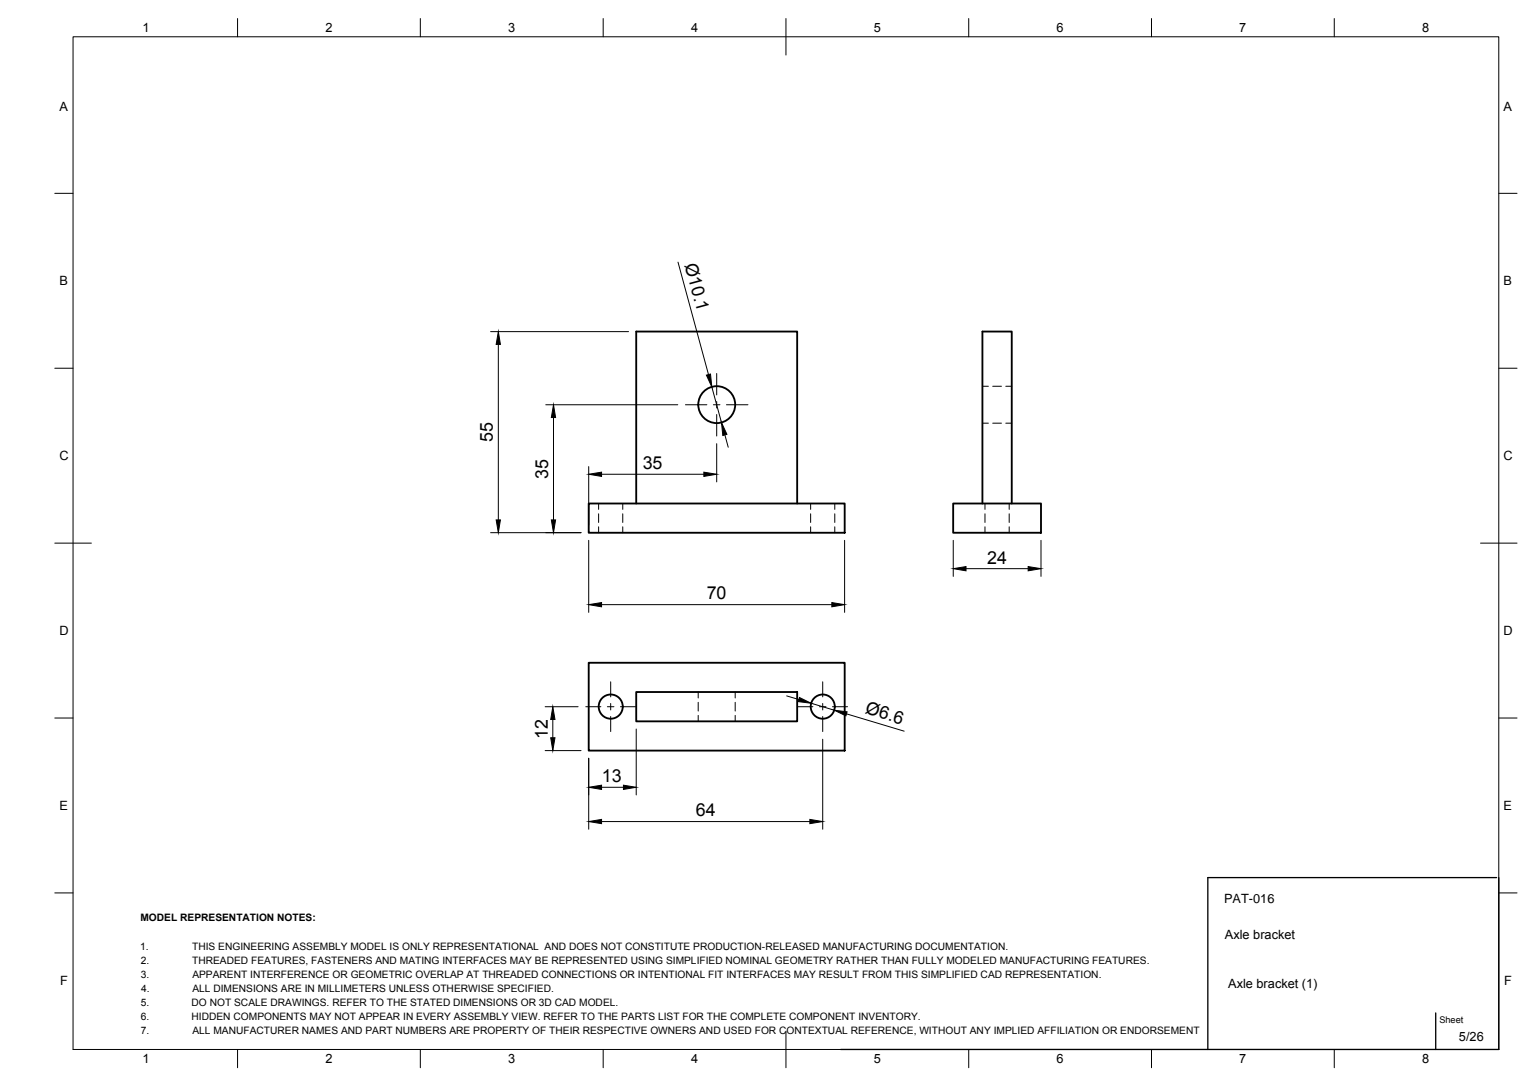
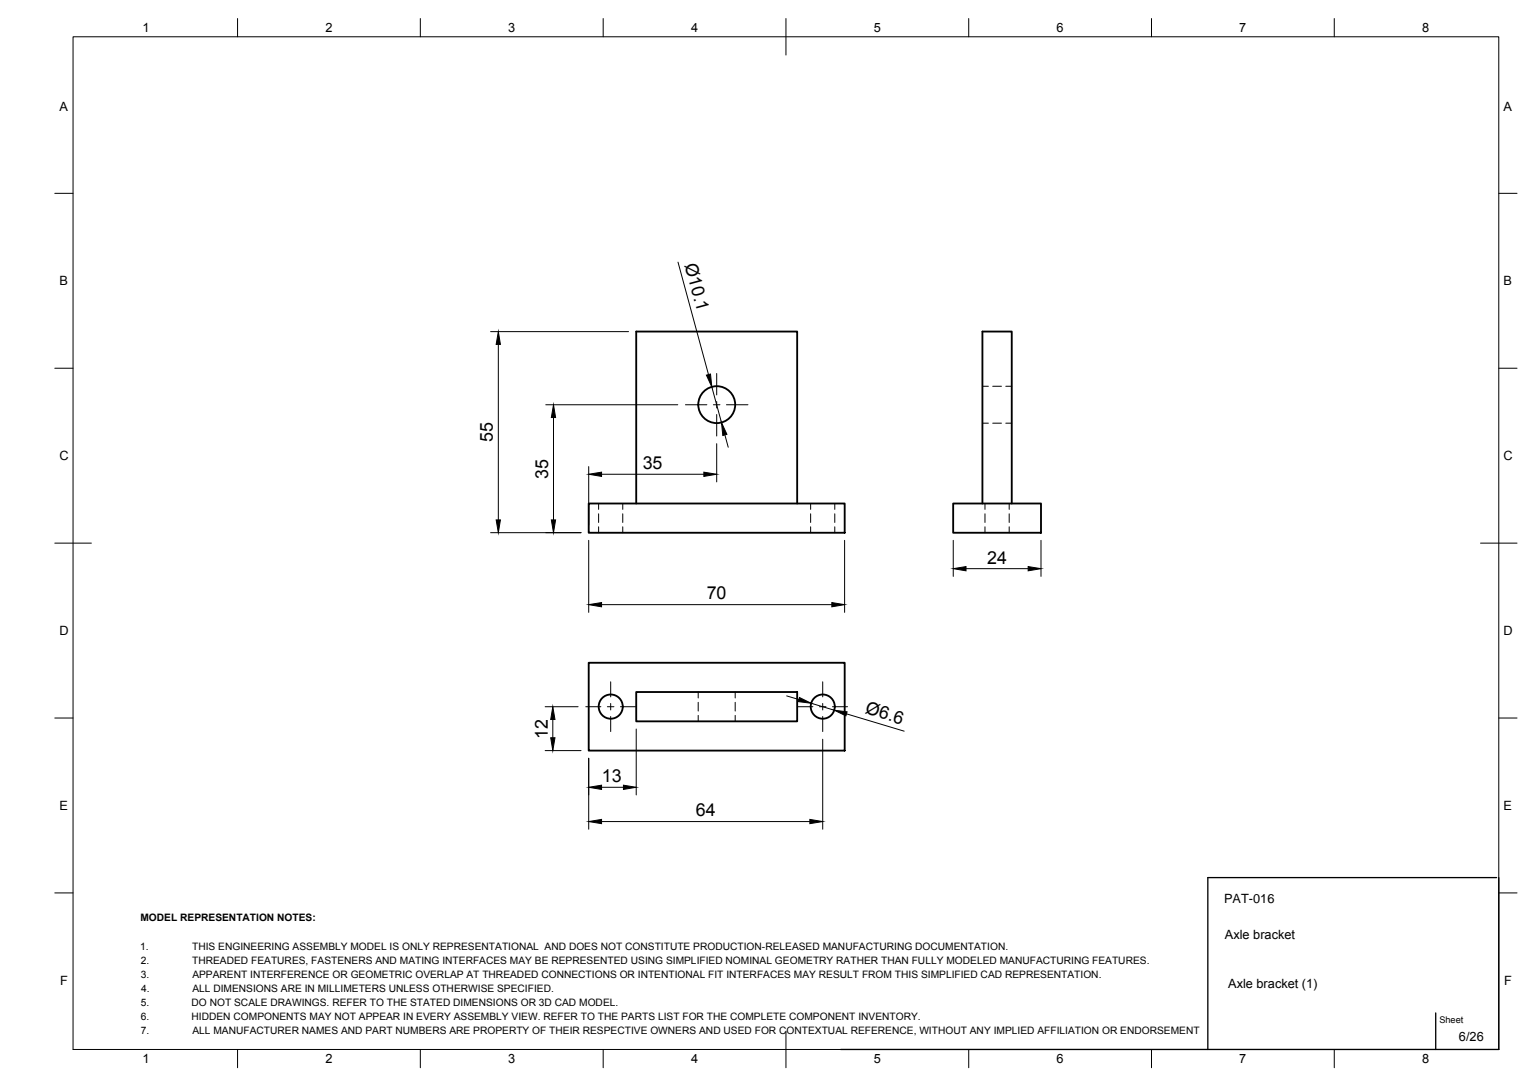
ISO-10303-21;
HEADER;
/* Generated by software containing ST-Developer
 * from STEP Tools, Inc. (www.steptools.com) 
 */

FILE_DESCRIPTION(
/* description */ ('Bracket-mounted idler roller'),
/* implementation_level */ '2;1');

FILE_NAME(
/* name */ 'Axle bracket (1).step',
/* time_stamp */ '2026-10-28T03:26:42-07:00',
/* author */ (''),
/* organization */ (''),
/* preprocessor_version */ 'ST-DEVELOPER v20.2',
/* originating_system */ 'Autodesk Translation Framework v15.17.0.0',
/* authorisation */ '');

FILE_SCHEMA (('AUTOMOTIVE_DESIGN { 1 0 10303 214 3 1 1 }'));
ENDSEC;

DATA;
#10=MECHANICAL_DESIGN_GEOMETRIC_PRESENTATION_REPRESENTATION('',(#281),#6241);
#239=SHAPE_REPRESENTATION_RELATIONSHIP('SRR','None',#6343,#260);
#260=ADVANCED_BREP_SHAPE_REPRESENTATION('',(#310),#6219);
#281=STYLED_ITEM('',(#6538),#310);
#310=MANIFOLD_SOLID_BREP('Body1',#3183);
#343=FACE_BOUND('',#732,.T.);
#344=FACE_BOUND('',#733,.T.);
#345=FACE_BOUND('',#734,.T.);
#346=FACE_BOUND('',#740,.T.);
#347=FACE_BOUND('',#743,.T.);
#348=FACE_BOUND('',#747,.T.);
#349=FACE_BOUND('',#748,.T.);
#428=PLANE('',#3478);
#429=PLANE('',#3479);
#430=PLANE('',#3480);
#431=PLANE('',#3481);
#432=PLANE('',#3482);
#433=PLANE('',#3483);
#434=PLANE('',#3484);
#435=PLANE('',#3485);
#436=PLANE('',#3486);
#437=PLANE('',#3487);
#438=PLANE('',#3488);
#530=FACE_OUTER_BOUND('',#728,.T.);
#531=FACE_OUTER_BOUND('',#729,.T.);
#532=FACE_OUTER_BOUND('',#730,.T.);
#533=FACE_OUTER_BOUND('',#731,.T.);
#534=FACE_OUTER_BOUND('',#735,.T.);
#535=FACE_OUTER_BOUND('',#736,.T.);
#536=FACE_OUTER_BOUND('',#737,.T.);
#537=FACE_OUTER_BOUND('',#738,.T.);
#538=FACE_OUTER_BOUND('',#739,.T.);
#539=FACE_OUTER_BOUND('',#741,.T.);
#540=FACE_OUTER_BOUND('',#742,.T.);
#541=FACE_OUTER_BOUND('',#744,.T.);
#542=FACE_OUTER_BOUND('',#745,.T.);
#543=FACE_OUTER_BOUND('',#746,.T.);
#728=EDGE_LOOP('',(#2232,#2233,#2234,#2235));
#729=EDGE_LOOP('',(#2236,#2237,#2238,#2239));
#730=EDGE_LOOP('',(#2240,#2241,#2242,#2243));
#731=EDGE_LOOP('',(#2244,#2245,#2246,#2247));
#732=EDGE_LOOP('',(#2248));
#733=EDGE_LOOP('',(#2249));
#734=EDGE_LOOP('',(#2250,#2251,#2252,#2253));
#735=EDGE_LOOP('',(#2254,#2255,#2256,#2257));
#736=EDGE_LOOP('',(#2258,#2259,#2260,#2261));
#737=EDGE_LOOP('',(#2262,#2263,#2264,#2265));
#738=EDGE_LOOP('',(#2266,#2267,#2268,#2269));
#739=EDGE_LOOP('',(#2270,#2271,#2272,#2273));
#740=EDGE_LOOP('',(#2274));
#741=EDGE_LOOP('',(#2275,#2276,#2277,#2278));
#742=EDGE_LOOP('',(#2279,#2280,#2281,#2282));
#743=EDGE_LOOP('',(#2283));
#744=EDGE_LOOP('',(#2284,#2285,#2286,#2287));
#745=EDGE_LOOP('',(#2288,#2289,#2290,#2291));
#746=EDGE_LOOP('',(#2292,#2293,#2294,#2295));
#747=EDGE_LOOP('',(#2296));
#748=EDGE_LOOP('',(#2297));
#1006=LINE('',#5027,#1188);
#1007=LINE('',#5033,#1189);
#1008=LINE('',#5039,#1190);
#1009=LINE('',#5044,#1191);
#1010=LINE('',#5046,#1192);
#1011=LINE('',#5048,#1193);
#1012=LINE('',#5049,#1194);
#1013=LINE('',#5052,#1195);
#1014=LINE('',#5054,#1196);
#1015=LINE('',#5056,#1197);
#1016=LINE('',#5057,#1198);
#1017=LINE('',#5060,#1199);
#1018=LINE('',#5062,#1200);
#1019=LINE('',#5063,#1201);
#1020=LINE('',#5066,#1202);
#1021=LINE('',#5068,#1203);
#1022=LINE('',#5069,#1204);
#1023=LINE('',#5071,#1205);
#1024=LINE('',#5073,#1206);
#1025=LINE('',#5076,#1207);
#1026=LINE('',#5078,#1208);
#1027=LINE('',#5079,#1209);
#1028=LINE('',#5082,#1210);
#1029=LINE('',#5083,#1211);
#1030=LINE('',#5086,#1212);
#1031=LINE('',#5087,#1213);
#1032=LINE('',#5089,#1214);
#1188=VECTOR('',#3965,0.33);
#1189=VECTOR('',#3972,0.33);
#1190=VECTOR('',#3979,0.505);
#1191=VECTOR('',#3984,1.);
#1192=VECTOR('',#3985,1.);
#1193=VECTOR('',#3986,1.);
#1194=VECTOR('',#3987,1.);
#1195=VECTOR('',#3988,1.);
#1196=VECTOR('',#3989,1.);
#1197=VECTOR('',#3990,1.);
#1198=VECTOR('',#3991,1.);
#1199=VECTOR('',#3994,1.);
#1200=VECTOR('',#3995,1.);
#1201=VECTOR('',#3996,1.);
#1202=VECTOR('',#3999,1.);
#1203=VECTOR('',#4000,1.);
#1204=VECTOR('',#4001,1.);
#1205=VECTOR('',#4004,1.);
#1206=VECTOR('',#4007,1.);
#1207=VECTOR('',#4010,1.);
#1208=VECTOR('',#4011,1.);
#1209=VECTOR('',#4012,1.);
#1210=VECTOR('',#4015,1.);
#1211=VECTOR('',#4016,1.);
#1212=VECTOR('',#4019,1.);
#1213=VECTOR('',#4020,1.);
#1214=VECTOR('',#4023,1.);
#1349=CIRCLE('',#3470,0.33);
#1350=CIRCLE('',#3471,0.33);
#1351=CIRCLE('',#3473,0.33);
#1352=CIRCLE('',#3474,0.33);
#1353=CIRCLE('',#3476,0.505);
#1354=CIRCLE('',#3477,0.505);
#1546=VERTEX_POINT('',#5024);
#1547=VERTEX_POINT('',#5026);
#1548=VERTEX_POINT('',#5030);
#1549=VERTEX_POINT('',#5032);
#1550=VERTEX_POINT('',#5036);
#1551=VERTEX_POINT('',#5038);
#1552=VERTEX_POINT('',#5042);
#1553=VERTEX_POINT('',#5043);
#1554=VERTEX_POINT('',#5045);
#1555=VERTEX_POINT('',#5047);
#1556=VERTEX_POINT('',#5050);
#1557=VERTEX_POINT('',#5051);
#1558=VERTEX_POINT('',#5053);
#1559=VERTEX_POINT('',#5055);
#1560=VERTEX_POINT('',#5059);
#1561=VERTEX_POINT('',#5061);
#1562=VERTEX_POINT('',#5065);
#1563=VERTEX_POINT('',#5067);
#1564=VERTEX_POINT('',#5075);
#1565=VERTEX_POINT('',#5077);
#1566=VERTEX_POINT('',#5081);
#1567=VERTEX_POINT('',#5085);
#1818=EDGE_CURVE('',#1546,#1546,#1349,.T.);
#1819=EDGE_CURVE('',#1546,#1547,#1006,.T.);
#1820=EDGE_CURVE('',#1547,#1547,#1350,.T.);
#1821=EDGE_CURVE('',#1548,#1548,#1351,.T.);
#1822=EDGE_CURVE('',#1548,#1549,#1007,.T.);
#1823=EDGE_CURVE('',#1549,#1549,#1352,.T.);
#1824=EDGE_CURVE('',#1550,#1550,#1353,.T.);
#1825=EDGE_CURVE('',#1550,#1551,#1008,.T.);
#1826=EDGE_CURVE('',#1551,#1551,#1354,.T.);
#1827=EDGE_CURVE('',#1552,#1553,#1009,.T.);
#1828=EDGE_CURVE('',#1552,#1554,#1010,.T.);
#1829=EDGE_CURVE('',#1555,#1554,#1011,.T.);
#1830=EDGE_CURVE('',#1553,#1555,#1012,.T.);
#1831=EDGE_CURVE('',#1556,#1557,#1013,.T.);
#1832=EDGE_CURVE('',#1558,#1556,#1014,.T.);
#1833=EDGE_CURVE('',#1559,#1558,#1015,.T.);
#1834=EDGE_CURVE('',#1557,#1559,#1016,.T.);
#1835=EDGE_CURVE('',#1553,#1560,#1017,.T.);
#1836=EDGE_CURVE('',#1561,#1555,#1018,.T.);
#1837=EDGE_CURVE('',#1560,#1561,#1019,.T.);
#1838=EDGE_CURVE('',#1562,#1552,#1020,.T.);
#1839=EDGE_CURVE('',#1562,#1563,#1021,.T.);
#1840=EDGE_CURVE('',#1554,#1563,#1022,.T.);
#1841=EDGE_CURVE('',#1563,#1561,#1023,.T.);
#1842=EDGE_CURVE('',#1560,#1562,#1024,.T.);
#1843=EDGE_CURVE('',#1558,#1564,#1025,.T.);
#1844=EDGE_CURVE('',#1565,#1564,#1026,.T.);
#1845=EDGE_CURVE('',#1559,#1565,#1027,.T.);
#1846=EDGE_CURVE('',#1556,#1566,#1028,.T.);
#1847=EDGE_CURVE('',#1564,#1566,#1029,.T.);
#1848=EDGE_CURVE('',#1557,#1567,#1030,.T.);
#1849=EDGE_CURVE('',#1566,#1567,#1031,.T.);
#1850=EDGE_CURVE('',#1567,#1565,#1032,.T.);
#2232=ORIENTED_EDGE('',*,*,#1818,.F.);
#2233=ORIENTED_EDGE('',*,*,#1819,.T.);
#2234=ORIENTED_EDGE('',*,*,#1820,.F.);
#2235=ORIENTED_EDGE('',*,*,#1819,.F.);
#2236=ORIENTED_EDGE('',*,*,#1821,.F.);
#2237=ORIENTED_EDGE('',*,*,#1822,.T.);
#2238=ORIENTED_EDGE('',*,*,#1823,.F.);
#2239=ORIENTED_EDGE('',*,*,#1822,.F.);
#2240=ORIENTED_EDGE('',*,*,#1824,.F.);
#2241=ORIENTED_EDGE('',*,*,#1825,.T.);
#2242=ORIENTED_EDGE('',*,*,#1826,.F.);
#2243=ORIENTED_EDGE('',*,*,#1825,.F.);
#2244=ORIENTED_EDGE('',*,*,#1827,.F.);
#2245=ORIENTED_EDGE('',*,*,#1828,.T.);
#2246=ORIENTED_EDGE('',*,*,#1829,.F.);
#2247=ORIENTED_EDGE('',*,*,#1830,.F.);
#2248=ORIENTED_EDGE('',*,*,#1820,.T.);
#2249=ORIENTED_EDGE('',*,*,#1823,.T.);
#2250=ORIENTED_EDGE('',*,*,#1831,.F.);
#2251=ORIENTED_EDGE('',*,*,#1832,.F.);
#2252=ORIENTED_EDGE('',*,*,#1833,.F.);
#2253=ORIENTED_EDGE('',*,*,#1834,.F.);
#2254=ORIENTED_EDGE('',*,*,#1835,.F.);
#2255=ORIENTED_EDGE('',*,*,#1830,.T.);
#2256=ORIENTED_EDGE('',*,*,#1836,.F.);
#2257=ORIENTED_EDGE('',*,*,#1837,.F.);
#2258=ORIENTED_EDGE('',*,*,#1838,.F.);
#2259=ORIENTED_EDGE('',*,*,#1839,.T.);
#2260=ORIENTED_EDGE('',*,*,#1840,.F.);
#2261=ORIENTED_EDGE('',*,*,#1828,.F.);
#2262=ORIENTED_EDGE('',*,*,#1829,.T.);
#2263=ORIENTED_EDGE('',*,*,#1840,.T.);
#2264=ORIENTED_EDGE('',*,*,#1841,.T.);
#2265=ORIENTED_EDGE('',*,*,#1836,.T.);
#2266=ORIENTED_EDGE('',*,*,#1827,.T.);
#2267=ORIENTED_EDGE('',*,*,#1835,.T.);
#2268=ORIENTED_EDGE('',*,*,#1842,.T.);
#2269=ORIENTED_EDGE('',*,*,#1838,.T.);
#2270=ORIENTED_EDGE('',*,*,#1833,.T.);
#2271=ORIENTED_EDGE('',*,*,#1843,.T.);
#2272=ORIENTED_EDGE('',*,*,#1844,.F.);
#2273=ORIENTED_EDGE('',*,*,#1845,.F.);
#2274=ORIENTED_EDGE('',*,*,#1824,.T.);
#2275=ORIENTED_EDGE('',*,*,#1832,.T.);
#2276=ORIENTED_EDGE('',*,*,#1846,.T.);
#2277=ORIENTED_EDGE('',*,*,#1847,.F.);
#2278=ORIENTED_EDGE('',*,*,#1843,.F.);
#2279=ORIENTED_EDGE('',*,*,#1831,.T.);
#2280=ORIENTED_EDGE('',*,*,#1848,.T.);
#2281=ORIENTED_EDGE('',*,*,#1849,.F.);
#2282=ORIENTED_EDGE('',*,*,#1846,.F.);
#2283=ORIENTED_EDGE('',*,*,#1826,.T.);
#2284=ORIENTED_EDGE('',*,*,#1834,.T.);
#2285=ORIENTED_EDGE('',*,*,#1845,.T.);
#2286=ORIENTED_EDGE('',*,*,#1850,.F.);
#2287=ORIENTED_EDGE('',*,*,#1848,.F.);
#2288=ORIENTED_EDGE('',*,*,#1850,.T.);
#2289=ORIENTED_EDGE('',*,*,#1844,.T.);
#2290=ORIENTED_EDGE('',*,*,#1847,.T.);
#2291=ORIENTED_EDGE('',*,*,#1849,.T.);
#2292=ORIENTED_EDGE('',*,*,#1842,.F.);
#2293=ORIENTED_EDGE('',*,*,#1837,.T.);
#2294=ORIENTED_EDGE('',*,*,#1841,.F.);
#2295=ORIENTED_EDGE('',*,*,#1839,.F.);
#2296=ORIENTED_EDGE('',*,*,#1818,.T.);
#2297=ORIENTED_EDGE('',*,*,#1821,.T.);
#2931=CYLINDRICAL_SURFACE('',#3469,0.33);
#2932=CYLINDRICAL_SURFACE('',#3472,0.33);
#2933=CYLINDRICAL_SURFACE('',#3475,0.505);
#3005=ADVANCED_FACE('',(#530),#2931,.F.);
#3006=ADVANCED_FACE('',(#531),#2932,.F.);
#3007=ADVANCED_FACE('',(#532),#2933,.F.);
#3008=ADVANCED_FACE('',(#533,#343,#344,#345),#428,.T.);
#3009=ADVANCED_FACE('',(#534),#429,.T.);
#3010=ADVANCED_FACE('',(#535),#430,.T.);
#3011=ADVANCED_FACE('',(#536),#431,.T.);
#3012=ADVANCED_FACE('',(#537),#432,.F.);
#3013=ADVANCED_FACE('',(#538,#346),#433,.T.);
#3014=ADVANCED_FACE('',(#539),#434,.T.);
#3015=ADVANCED_FACE('',(#540,#347),#435,.T.);
#3016=ADVANCED_FACE('',(#541),#436,.T.);
#3017=ADVANCED_FACE('',(#542),#437,.T.);
#3018=ADVANCED_FACE('',(#543,#348,#349),#438,.F.);
#3183=CLOSED_SHELL('',(#3005,#3006,#3007,#3008,#3009,#3010,#3011,#3012,
#3013,#3014,#3015,#3016,#3017,#3018));
#3468=AXIS2_PLACEMENT_3D('',#5022,#3959,#3960);
#3469=AXIS2_PLACEMENT_3D('',#5023,#3961,#3962);
#3470=AXIS2_PLACEMENT_3D('',#5025,#3963,#3964);
#3471=AXIS2_PLACEMENT_3D('',#5028,#3966,#3967);
#3472=AXIS2_PLACEMENT_3D('',#5029,#3968,#3969);
#3473=AXIS2_PLACEMENT_3D('',#5031,#3970,#3971);
#3474=AXIS2_PLACEMENT_3D('',#5034,#3973,#3974);
#3475=AXIS2_PLACEMENT_3D('',#5035,#3975,#3976);
#3476=AXIS2_PLACEMENT_3D('',#5037,#3977,#3978);
#3477=AXIS2_PLACEMENT_3D('',#5040,#3980,#3981);
#3478=AXIS2_PLACEMENT_3D('',#5041,#3982,#3983);
#3479=AXIS2_PLACEMENT_3D('',#5058,#3992,#3993);
#3480=AXIS2_PLACEMENT_3D('',#5064,#3997,#3998);
#3481=AXIS2_PLACEMENT_3D('',#5070,#4002,#4003);
#3482=AXIS2_PLACEMENT_3D('',#5072,#4005,#4006);
#3483=AXIS2_PLACEMENT_3D('',#5074,#4008,#4009);
#3484=AXIS2_PLACEMENT_3D('',#5080,#4013,#4014);
#3485=AXIS2_PLACEMENT_3D('',#5084,#4017,#4018);
#3486=AXIS2_PLACEMENT_3D('',#5088,#4021,#4022);
#3487=AXIS2_PLACEMENT_3D('',#5090,#4024,#4025);
#3488=AXIS2_PLACEMENT_3D('',#5091,#4026,#4027);
#3959=DIRECTION('axis',(0.,0.,1.));
#3960=DIRECTION('refdir',(1.,0.,0.));
#3961=DIRECTION('center_axis',(0.,0.,1.));
#3962=DIRECTION('ref_axis',(1.,0.,0.));
#3963=DIRECTION('center_axis',(0.,0.,1.));
#3964=DIRECTION('ref_axis',(1.,0.,0.));
#3965=DIRECTION('',(0.,0.,1.));
#3966=DIRECTION('center_axis',(0.,0.,-1.));
#3967=DIRECTION('ref_axis',(1.,0.,0.));
#3968=DIRECTION('center_axis',(0.,0.,1.));
#3969=DIRECTION('ref_axis',(1.,0.,0.));
#3970=DIRECTION('center_axis',(0.,0.,1.));
#3971=DIRECTION('ref_axis',(1.,0.,0.));
#3972=DIRECTION('',(0.,0.,1.));
#3973=DIRECTION('center_axis',(0.,0.,-1.));
#3974=DIRECTION('ref_axis',(1.,0.,0.));
#3975=DIRECTION('center_axis',(0.,1.,0.));
#3976=DIRECTION('ref_axis',(1.,0.,0.));
#3977=DIRECTION('center_axis',(0.,1.,0.));
#3978=DIRECTION('ref_axis',(1.,0.,0.));
#3979=DIRECTION('',(0.,1.,0.));
#3980=DIRECTION('center_axis',(0.,-1.,0.));
#3981=DIRECTION('ref_axis',(1.,0.,0.));
#3982=DIRECTION('center_axis',(0.,0.,1.));
#3983=DIRECTION('ref_axis',(1.,0.,0.));
#3984=DIRECTION('',(-1.,0.,0.));
#3985=DIRECTION('',(0.,1.,0.));
#3986=DIRECTION('',(1.,0.,0.));
#3987=DIRECTION('',(0.,1.,0.));
#3988=DIRECTION('',(-1.,0.,0.));
#3989=DIRECTION('',(0.,1.,0.));
#3990=DIRECTION('',(1.,0.,0.));
#3991=DIRECTION('',(0.,-1.,0.));
#3992=DIRECTION('center_axis',(-1.,0.,0.));
#3993=DIRECTION('ref_axis',(0.,0.,1.));
#3994=DIRECTION('',(0.,0.,-1.));
#3995=DIRECTION('',(0.,0.,1.));
#3996=DIRECTION('',(0.,1.,0.));
#3997=DIRECTION('center_axis',(1.,0.,0.));
#3998=DIRECTION('ref_axis',(0.,0.,-1.));
#3999=DIRECTION('',(0.,0.,1.));
#4000=DIRECTION('',(0.,1.,0.));
#4001=DIRECTION('',(0.,0.,-1.));
#4002=DIRECTION('center_axis',(0.,1.,0.));
#4003=DIRECTION('ref_axis',(0.,0.,1.));
#4004=DIRECTION('',(-1.,0.,0.));
#4005=DIRECTION('center_axis',(0.,1.,0.));
#4006=DIRECTION('ref_axis',(1.,0.,0.));
#4007=DIRECTION('',(1.,0.,0.));
#4008=DIRECTION('center_axis',(0.,-1.,0.));
#4009=DIRECTION('ref_axis',(1.,0.,0.));
#4010=DIRECTION('',(0.,0.,1.));
#4011=DIRECTION('',(1.,0.,0.));
#4012=DIRECTION('',(0.,0.,1.));
#4013=DIRECTION('center_axis',(1.,0.,0.));
#4014=DIRECTION('ref_axis',(0.,1.,0.));
#4015=DIRECTION('',(0.,0.,1.));
#4016=DIRECTION('',(0.,1.,0.));
#4017=DIRECTION('center_axis',(0.,1.,0.));
#4018=DIRECTION('ref_axis',(-1.,0.,0.));
#4019=DIRECTION('',(0.,0.,1.));
#4020=DIRECTION('',(-1.,0.,0.));
#4021=DIRECTION('center_axis',(-1.,0.,0.));
#4022=DIRECTION('ref_axis',(0.,-1.,0.));
#4023=DIRECTION('',(0.,-1.,0.));
#4024=DIRECTION('center_axis',(0.,0.,1.));
#4025=DIRECTION('ref_axis',(1.,0.,0.));
#4026=DIRECTION('center_axis',(0.,0.,1.));
#4027=DIRECTION('ref_axis',(1.,0.,0.));
#5022=CARTESIAN_POINT('',(0.,0.,0.));
#5023=CARTESIAN_POINT('Origin',(-2.9,32.,0.9));
#5024=CARTESIAN_POINT('',(-3.23,32.,1.));
#5025=CARTESIAN_POINT('Origin',(-2.9,32.,1.));
#5026=CARTESIAN_POINT('',(-3.23,32.,1.8));
#5027=CARTESIAN_POINT('',(-3.23,32.,0.9));
#5028=CARTESIAN_POINT('Origin',(-2.9,32.,1.8));
#5029=CARTESIAN_POINT('Origin',(2.9,32.,0.9));
#5030=CARTESIAN_POINT('',(2.57,32.,1.));
#5031=CARTESIAN_POINT('Origin',(2.9,32.,1.));
#5032=CARTESIAN_POINT('',(2.57,32.,1.8));
#5033=CARTESIAN_POINT('',(2.57,32.,0.9));
#5034=CARTESIAN_POINT('Origin',(2.9,32.,1.8));
#5035=CARTESIAN_POINT('Origin',(0.,31.5,4.5));
#5036=CARTESIAN_POINT('',(-0.505,31.6,4.5));
#5037=CARTESIAN_POINT('Origin',(0.,31.6,4.5));
#5038=CARTESIAN_POINT('',(-0.505,32.4,4.5));
#5039=CARTESIAN_POINT('',(-0.505,31.5,4.5));
#5040=CARTESIAN_POINT('Origin',(0.,32.4,4.5));
#5041=CARTESIAN_POINT('Origin',(-3.5,30.8,1.8));
#5042=CARTESIAN_POINT('',(3.5,30.8,1.8));
#5043=CARTESIAN_POINT('',(-3.5,30.8,1.8));
#5044=CARTESIAN_POINT('',(3.5,30.8,1.8));
#5045=CARTESIAN_POINT('',(3.5,33.2,1.8));
#5046=CARTESIAN_POINT('',(3.5,30.8,1.8));
#5047=CARTESIAN_POINT('',(-3.5,33.2,1.8));
#5048=CARTESIAN_POINT('',(3.5,33.2,1.8));
#5049=CARTESIAN_POINT('',(-3.5,30.8,1.8));
#5050=CARTESIAN_POINT('',(2.2,32.4,1.8));
#5051=CARTESIAN_POINT('',(-2.2,32.4,1.8));
#5052=CARTESIAN_POINT('',(-0.65,32.4,1.8));
#5053=CARTESIAN_POINT('',(2.2,31.6,1.8));
#5054=CARTESIAN_POINT('',(2.2,31.2,1.8));
#5055=CARTESIAN_POINT('',(-2.2,31.6,1.8));
#5056=CARTESIAN_POINT('',(-2.85,31.6,1.8));
#5057=CARTESIAN_POINT('',(-2.2,31.6,1.8));
#5058=CARTESIAN_POINT('Origin',(-3.5,30.8,1.));
#5059=CARTESIAN_POINT('',(-3.5,30.8,1.));
#5060=CARTESIAN_POINT('',(-3.5,30.8,1.8));
#5061=CARTESIAN_POINT('',(-3.5,33.2,1.));
#5062=CARTESIAN_POINT('',(-3.5,33.2,1.8));
#5063=CARTESIAN_POINT('',(-3.5,30.8,1.));
#5064=CARTESIAN_POINT('Origin',(3.5,30.8,1.8));
#5065=CARTESIAN_POINT('',(3.5,30.8,1.));
#5066=CARTESIAN_POINT('',(3.5,30.8,1.));
#5067=CARTESIAN_POINT('',(3.5,33.2,1.));
#5068=CARTESIAN_POINT('',(3.5,30.8,1.));
#5069=CARTESIAN_POINT('',(3.5,33.2,1.));
#5070=CARTESIAN_POINT('Origin',(0.,33.2,1.4));
#5071=CARTESIAN_POINT('',(-3.5,33.2,1.));
#5072=CARTESIAN_POINT('Origin',(0.,30.8,1.4));
#5073=CARTESIAN_POINT('',(-3.5,30.8,1.));
#5074=CARTESIAN_POINT('Origin',(-2.2,31.6,1.));
#5075=CARTESIAN_POINT('',(2.2,31.6,6.5));
#5076=CARTESIAN_POINT('',(2.2,31.6,1.));
#5077=CARTESIAN_POINT('',(-2.2,31.6,6.5));
#5078=CARTESIAN_POINT('',(-2.2,31.6,6.5));
#5079=CARTESIAN_POINT('',(-2.2,31.6,1.));
#5080=CARTESIAN_POINT('Origin',(2.2,31.6,1.));
#5081=CARTESIAN_POINT('',(2.2,32.4,6.5));
#5082=CARTESIAN_POINT('',(2.2,32.4,1.));
#5083=CARTESIAN_POINT('',(2.2,31.6,6.5));
#5084=CARTESIAN_POINT('Origin',(2.2,32.4,1.));
#5085=CARTESIAN_POINT('',(-2.2,32.4,6.5));
#5086=CARTESIAN_POINT('',(-2.2,32.4,1.));
#5087=CARTESIAN_POINT('',(2.2,32.4,6.5));
#5088=CARTESIAN_POINT('Origin',(-2.2,32.4,1.));
#5089=CARTESIAN_POINT('',(-2.2,32.4,6.5));
#5090=CARTESIAN_POINT('Origin',(0.,32.,6.5));
#5091=CARTESIAN_POINT('Origin',(0.,32.,1.));
#6193=UNCERTAINTY_MEASURE_WITH_UNIT(LENGTH_MEASURE(0.001),#6242,
'DISTANCE_ACCURACY_VALUE',
'Maximum model space distance between geometric entities at asserted c
onnectivities');
#6215=UNCERTAINTY_MEASURE_WITH_UNIT(LENGTH_MEASURE(0.001),#6242,
'DISTANCE_ACCURACY_VALUE',
'Maximum model space distance between geometric entities at asserted c
onnectivities');
#6219=(
GEOMETRIC_REPRESENTATION_CONTEXT(3)
GLOBAL_UNCERTAINTY_ASSIGNED_CONTEXT((#6193))
GLOBAL_UNIT_ASSIGNED_CONTEXT((#6242,#6244,#6245))
REPRESENTATION_CONTEXT('','3D')
);
#6241=(
GEOMETRIC_REPRESENTATION_CONTEXT(3)
GLOBAL_UNCERTAINTY_ASSIGNED_CONTEXT((#6215))
GLOBAL_UNIT_ASSIGNED_CONTEXT((#6242,#6244,#6245))
REPRESENTATION_CONTEXT('','3D')
);
#6242=(
LENGTH_UNIT()
NAMED_UNIT(*)
SI_UNIT(.CENTI.,.METRE.)
);
#6244=(
NAMED_UNIT(*)
PLANE_ANGLE_UNIT()
SI_UNIT($,.RADIAN.)
);
#6245=(
NAMED_UNIT(*)
SI_UNIT($,.STERADIAN.)
SOLID_ANGLE_UNIT()
);
#6249=SHAPE_DEFINITION_REPRESENTATION(#6274,#6343);
#6274=PRODUCT_DEFINITION_SHAPE('',$,#6369);
#6343=SHAPE_REPRESENTATION('',(#3468),#6219);
#6365=PRODUCT_DEFINITION_CONTEXT('part definition',#6442,'design');
#6369=PRODUCT_DEFINITION('Axle bracket (1)','Axle bracket (1)',#6394,#6365);
#6394=PRODUCT_DEFINITION_FORMATION('',$,#6447);
#6442=APPLICATION_CONTEXT(
'Core Data for Automotive Mechanical Design Process');
#6443=PRODUCT_CONTEXT('part definition',#6442,'mechanical');
#6447=PRODUCT('Axle bracket (1)','Axle bracket (1)','Axle bracket (1)',(#6443));
#6532=COLOUR_RGB('Grey',0.48,0.52,0.57);
#6533=FILL_AREA_STYLE_COLOUR('',#6532);
#6534=FILL_AREA_STYLE('',(#6533));
#6535=SURFACE_STYLE_FILL_AREA(#6534);
#6536=SURFACE_SIDE_STYLE('',(#6535));
#6537=SURFACE_STYLE_USAGE(.BOTH.,#6536);
#6538=PRESENTATION_STYLE_ASSIGNMENT((#6537));
ENDSEC;
END-ISO-10303-21;
